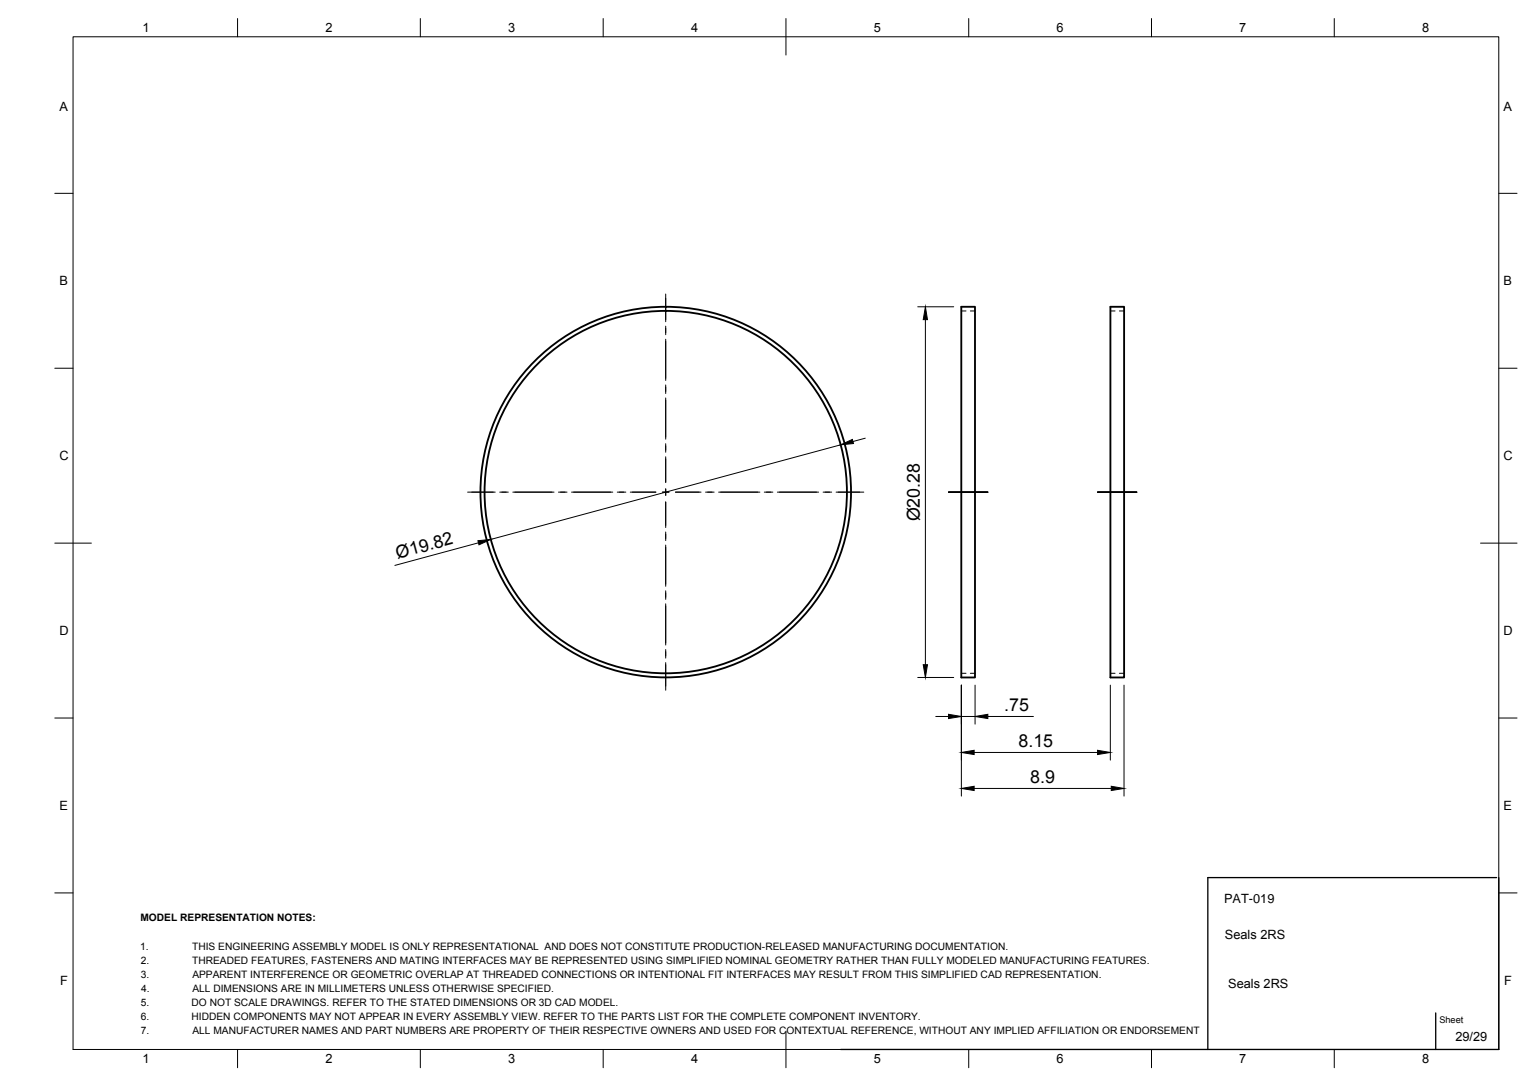
ISO-10303-21;
HEADER;
/* Generated by software containing ST-Developer
 * from STEP Tools, Inc. (www.steptools.com) 
 */

FILE_DESCRIPTION(
/* description */ ('Caster wheel assembly'),
/* implementation_level */ '2;1');

FILE_NAME(
/* name */ 'Seals 2RS.step',
/* time_stamp */ '2026-10-28T03:23:56-07:00',
/* author */ (''),
/* organization */ (''),
/* preprocessor_version */ 'ST-DEVELOPER v20.2',
/* originating_system */ 'Autodesk Translation Framework v15.17.0.0',
/* authorisation */ '');

FILE_SCHEMA (('AUTOMOTIVE_DESIGN { 1 0 10303 214 3 1 1 }'));
ENDSEC;

DATA;
#10=MECHANICAL_DESIGN_GEOMETRIC_PRESENTATION_REPRESENTATION('',(#250,#251),#5385);
#199=SHAPE_REPRESENTATION_RELATIONSHIP('SRR','None',#5497,#221);
#221=ADVANCED_BREP_SHAPE_REPRESENTATION('',(#279,#280),#5384);
#250=STYLED_ITEM('',(#5672),#279);
#251=STYLED_ITEM('',(#5672),#280);
#279=MANIFOLD_SOLID_BREP('Body1',#2678);
#280=MANIFOLD_SOLID_BREP('Body2',#2679);
#329=FACE_BOUND('',#798,.T.);
#330=FACE_BOUND('',#801,.T.);
#331=FACE_BOUND('',#804,.T.);
#332=FACE_BOUND('',#807,.T.);
#417=PLANE('',#3275);
#418=PLANE('',#3280);
#419=PLANE('',#3283);
#420=PLANE('',#3288);
#581=FACE_OUTER_BOUND('',#797,.T.);
#582=FACE_OUTER_BOUND('',#799,.T.);
#583=FACE_OUTER_BOUND('',#800,.T.);
#584=FACE_OUTER_BOUND('',#802,.T.);
#585=FACE_OUTER_BOUND('',#803,.T.);
#586=FACE_OUTER_BOUND('',#805,.T.);
#587=FACE_OUTER_BOUND('',#806,.T.);
#588=FACE_OUTER_BOUND('',#808,.T.);
#797=EDGE_LOOP('',(#2404));
#798=EDGE_LOOP('',(#2405));
#799=EDGE_LOOP('',(#2406,#2407,#2408,#2409));
#800=EDGE_LOOP('',(#2410));
#801=EDGE_LOOP('',(#2411));
#802=EDGE_LOOP('',(#2412,#2413,#2414,#2415));
#803=EDGE_LOOP('',(#2416));
#804=EDGE_LOOP('',(#2417));
#805=EDGE_LOOP('',(#2418,#2419,#2420,#2421));
#806=EDGE_LOOP('',(#2422));
#807=EDGE_LOOP('',(#2423));
#808=EDGE_LOOP('',(#2424,#2425,#2426,#2427));
#939=LINE('',#5297,#1073);
#940=LINE('',#5302,#1074);
#941=LINE('',#5311,#1075);
#942=LINE('',#5316,#1076);
#1073=VECTOR('',#4148,1.013815);
#1074=VECTOR('',#4155,0.991185);
#1075=VECTOR('',#4166,1.013815);
#1076=VECTOR('',#4173,0.991185);
#1228=CIRCLE('',#3276,1.013815);
#1229=CIRCLE('',#3277,0.991185);
#1230=CIRCLE('',#3279,1.013815);
#1231=CIRCLE('',#3281,0.991185);
#1232=CIRCLE('',#3284,1.013815);
#1233=CIRCLE('',#3285,0.991185);
#1234=CIRCLE('',#3287,1.013815);
#1235=CIRCLE('',#3289,0.991185);
#1451=VERTEX_POINT('',#5290);
#1452=VERTEX_POINT('',#5292);
#1453=VERTEX_POINT('',#5295);
#1454=VERTEX_POINT('',#5299);
#1455=VERTEX_POINT('',#5304);
#1456=VERTEX_POINT('',#5306);
#1457=VERTEX_POINT('',#5309);
#1458=VERTEX_POINT('',#5313);
#1770=EDGE_CURVE('',#1451,#1451,#1228,.T.);
#1771=EDGE_CURVE('',#1452,#1452,#1229,.T.);
#1772=EDGE_CURVE('',#1453,#1453,#1230,.T.);
#1773=EDGE_CURVE('',#1453,#1451,#939,.T.);
#1774=EDGE_CURVE('',#1454,#1454,#1231,.T.);
#1775=EDGE_CURVE('',#1454,#1452,#940,.T.);
#1776=EDGE_CURVE('',#1455,#1455,#1232,.T.);
#1777=EDGE_CURVE('',#1456,#1456,#1233,.T.);
#1778=EDGE_CURVE('',#1457,#1457,#1234,.T.);
#1779=EDGE_CURVE('',#1457,#1455,#941,.T.);
#1780=EDGE_CURVE('',#1458,#1458,#1235,.T.);
#1781=EDGE_CURVE('',#1458,#1456,#942,.T.);
#2404=ORIENTED_EDGE('',*,*,#1770,.F.);
#2405=ORIENTED_EDGE('',*,*,#1771,.T.);
#2406=ORIENTED_EDGE('',*,*,#1772,.F.);
#2407=ORIENTED_EDGE('',*,*,#1773,.T.);
#2408=ORIENTED_EDGE('',*,*,#1770,.T.);
#2409=ORIENTED_EDGE('',*,*,#1773,.F.);
#2410=ORIENTED_EDGE('',*,*,#1772,.T.);
#2411=ORIENTED_EDGE('',*,*,#1774,.F.);
#2412=ORIENTED_EDGE('',*,*,#1774,.T.);
#2413=ORIENTED_EDGE('',*,*,#1775,.T.);
#2414=ORIENTED_EDGE('',*,*,#1771,.F.);
#2415=ORIENTED_EDGE('',*,*,#1775,.F.);
#2416=ORIENTED_EDGE('',*,*,#1776,.F.);
#2417=ORIENTED_EDGE('',*,*,#1777,.T.);
#2418=ORIENTED_EDGE('',*,*,#1778,.F.);
#2419=ORIENTED_EDGE('',*,*,#1779,.T.);
#2420=ORIENTED_EDGE('',*,*,#1776,.T.);
#2421=ORIENTED_EDGE('',*,*,#1779,.F.);
#2422=ORIENTED_EDGE('',*,*,#1778,.T.);
#2423=ORIENTED_EDGE('',*,*,#1780,.F.);
#2424=ORIENTED_EDGE('',*,*,#1780,.T.);
#2425=ORIENTED_EDGE('',*,*,#1781,.T.);
#2426=ORIENTED_EDGE('',*,*,#1777,.F.);
#2427=ORIENTED_EDGE('',*,*,#1781,.F.);
#2477=CYLINDRICAL_SURFACE('',#3278,1.013815);
#2478=CYLINDRICAL_SURFACE('',#3282,0.991185);
#2479=CYLINDRICAL_SURFACE('',#3286,1.013815);
#2480=CYLINDRICAL_SURFACE('',#3290,0.991185);
#2641=ADVANCED_FACE('',(#581,#329),#417,.T.);
#2642=ADVANCED_FACE('',(#582),#2477,.T.);
#2643=ADVANCED_FACE('',(#583,#330),#418,.T.);
#2644=ADVANCED_FACE('',(#584),#2478,.F.);
#2645=ADVANCED_FACE('',(#585,#331),#419,.T.);
#2646=ADVANCED_FACE('',(#586),#2479,.T.);
#2647=ADVANCED_FACE('',(#587,#332),#420,.T.);
#2648=ADVANCED_FACE('',(#588),#2480,.F.);
#2678=CLOSED_SHELL('',(#2641,#2642,#2643,#2644));
#2679=CLOSED_SHELL('',(#2645,#2646,#2647,#2648));
#3274=AXIS2_PLACEMENT_3D('',#5288,#4136,#4137);
#3275=AXIS2_PLACEMENT_3D('',#5289,#4138,#4139);
#3276=AXIS2_PLACEMENT_3D('',#5291,#4140,#4141);
#3277=AXIS2_PLACEMENT_3D('',#5293,#4142,#4143);
#3278=AXIS2_PLACEMENT_3D('',#5294,#4144,#4145);
#3279=AXIS2_PLACEMENT_3D('',#5296,#4146,#4147);
#3280=AXIS2_PLACEMENT_3D('',#5298,#4149,#4150);
#3281=AXIS2_PLACEMENT_3D('',#5300,#4151,#4152);
#3282=AXIS2_PLACEMENT_3D('',#5301,#4153,#4154);
#3283=AXIS2_PLACEMENT_3D('',#5303,#4156,#4157);
#3284=AXIS2_PLACEMENT_3D('',#5305,#4158,#4159);
#3285=AXIS2_PLACEMENT_3D('',#5307,#4160,#4161);
#3286=AXIS2_PLACEMENT_3D('',#5308,#4162,#4163);
#3287=AXIS2_PLACEMENT_3D('',#5310,#4164,#4165);
#3288=AXIS2_PLACEMENT_3D('',#5312,#4167,#4168);
#3289=AXIS2_PLACEMENT_3D('',#5314,#4169,#4170);
#3290=AXIS2_PLACEMENT_3D('',#5315,#4171,#4172);
#4136=DIRECTION('axis',(0.,0.,1.));
#4137=DIRECTION('refdir',(1.,0.,0.));
#4138=DIRECTION('center_axis',(0.,1.,0.));
#4139=DIRECTION('ref_axis',(0.,0.,1.));
#4140=DIRECTION('center_axis',(0.,-1.,0.));
#4141=DIRECTION('ref_axis',(1.,0.,0.));
#4142=DIRECTION('center_axis',(0.,-1.,0.));
#4143=DIRECTION('ref_axis',(1.,0.,0.));
#4144=DIRECTION('center_axis',(0.,-1.,0.));
#4145=DIRECTION('ref_axis',(1.,0.,0.));
#4146=DIRECTION('center_axis',(0.,-1.,0.));
#4147=DIRECTION('ref_axis',(1.,0.,0.));
#4148=DIRECTION('',(0.,1.,0.));
#4149=DIRECTION('center_axis',(0.,-1.,0.));
#4150=DIRECTION('ref_axis',(0.,0.,-1.));
#4151=DIRECTION('center_axis',(0.,-1.,0.));
#4152=DIRECTION('ref_axis',(1.,0.,0.));
#4153=DIRECTION('center_axis',(0.,-1.,0.));
#4154=DIRECTION('ref_axis',(1.,0.,0.));
#4155=DIRECTION('',(0.,1.,0.));
#4156=DIRECTION('center_axis',(0.,1.,0.));
#4157=DIRECTION('ref_axis',(0.,0.,1.));
#4158=DIRECTION('center_axis',(0.,-1.,0.));
#4159=DIRECTION('ref_axis',(1.,0.,0.));
#4160=DIRECTION('center_axis',(0.,-1.,0.));
#4161=DIRECTION('ref_axis',(1.,0.,0.));
#4162=DIRECTION('center_axis',(0.,-1.,0.));
#4163=DIRECTION('ref_axis',(1.,0.,0.));
#4164=DIRECTION('center_axis',(0.,-1.,0.));
#4165=DIRECTION('ref_axis',(1.,0.,0.));
#4166=DIRECTION('',(0.,1.,0.));
#4167=DIRECTION('center_axis',(0.,-1.,0.));
#4168=DIRECTION('ref_axis',(0.,0.,-1.));
#4169=DIRECTION('center_axis',(0.,-1.,0.));
#4170=DIRECTION('ref_axis',(1.,0.,0.));
#4171=DIRECTION('center_axis',(0.,-1.,0.));
#4172=DIRECTION('ref_axis',(1.,0.,0.));
#4173=DIRECTION('',(0.,1.,0.));
#5288=CARTESIAN_POINT('',(0.,0.,0.));
#5289=CARTESIAN_POINT('Origin',(1.013815,0.445,0.));
#5290=CARTESIAN_POINT('',(-1.013815,0.445,-1.24156529467757E-16));
#5291=CARTESIAN_POINT('Origin',(0.,0.445,0.));
#5292=CARTESIAN_POINT('',(-0.991185,0.445,-1.21385153761287E-16));
#5293=CARTESIAN_POINT('Origin',(0.,0.445,0.));
#5294=CARTESIAN_POINT('Origin',(0.,0.4075,0.));
#5295=CARTESIAN_POINT('',(-1.013815,0.37,-1.24156529467757E-16));
#5296=CARTESIAN_POINT('Origin',(0.,0.37,0.));
#5297=CARTESIAN_POINT('',(-1.013815,0.4075,-1.24156529467757E-16));
#5298=CARTESIAN_POINT('Origin',(0.991185,0.37,0.));
#5299=CARTESIAN_POINT('',(-0.991185,0.37,-1.21385153761287E-16));
#5300=CARTESIAN_POINT('Origin',(0.,0.37,0.));
#5301=CARTESIAN_POINT('Origin',(0.,0.4075,0.));
#5302=CARTESIAN_POINT('',(-0.991185,0.4075,-1.21385153761287E-16));
#5303=CARTESIAN_POINT('Origin',(1.013815,-0.37,0.));
#5304=CARTESIAN_POINT('',(-1.013815,-0.37,-1.24156529467757E-16));
#5305=CARTESIAN_POINT('Origin',(0.,-0.37,0.));
#5306=CARTESIAN_POINT('',(-0.991185,-0.37,-1.21385153761287E-16));
#5307=CARTESIAN_POINT('Origin',(0.,-0.37,0.));
#5308=CARTESIAN_POINT('Origin',(0.,-0.4075,0.));
#5309=CARTESIAN_POINT('',(-1.013815,-0.445,-1.24156529467757E-16));
#5310=CARTESIAN_POINT('Origin',(0.,-0.445,0.));
#5311=CARTESIAN_POINT('',(-1.013815,-0.4075,-1.24156529467757E-16));
#5312=CARTESIAN_POINT('Origin',(0.991185,-0.445,0.));
#5313=CARTESIAN_POINT('',(-0.991185,-0.445,-1.21385153761287E-16));
#5314=CARTESIAN_POINT('Origin',(0.,-0.445,0.));
#5315=CARTESIAN_POINT('Origin',(0.,-0.4075,0.));
#5316=CARTESIAN_POINT('',(-0.991185,-0.4075,-1.21385153761287E-16));
#5356=UNCERTAINTY_MEASURE_WITH_UNIT(LENGTH_MEASURE(0.001),#5386,
'DISTANCE_ACCURACY_VALUE',
'Maximum model space distance between geometric entities at asserted c
onnectivities');
#5357=UNCERTAINTY_MEASURE_WITH_UNIT(LENGTH_MEASURE(0.001),#5386,
'DISTANCE_ACCURACY_VALUE',
'Maximum model space distance between geometric entities at asserted c
onnectivities');
#5384=(
GEOMETRIC_REPRESENTATION_CONTEXT(3)
GLOBAL_UNCERTAINTY_ASSIGNED_CONTEXT((#5356))
GLOBAL_UNIT_ASSIGNED_CONTEXT((#5386,#5388,#5389))
REPRESENTATION_CONTEXT('','3D')
);
#5385=(
GEOMETRIC_REPRESENTATION_CONTEXT(3)
GLOBAL_UNCERTAINTY_ASSIGNED_CONTEXT((#5357))
GLOBAL_UNIT_ASSIGNED_CONTEXT((#5386,#5388,#5389))
REPRESENTATION_CONTEXT('','3D')
);
#5386=(
LENGTH_UNIT()
NAMED_UNIT(*)
SI_UNIT(.CENTI.,.METRE.)
);
#5388=(
NAMED_UNIT(*)
PLANE_ANGLE_UNIT()
SI_UNIT($,.RADIAN.)
);
#5389=(
NAMED_UNIT(*)
SI_UNIT($,.STERADIAN.)
SOLID_ANGLE_UNIT()
);
#5416=SHAPE_DEFINITION_REPRESENTATION(#5457,#5497);
#5457=PRODUCT_DEFINITION_SHAPE('',$,#5525);
#5497=SHAPE_REPRESENTATION('',(#3274),#5384);
#5498=PRODUCT_DEFINITION_CONTEXT('part definition',#5581,'design');
#5525=PRODUCT_DEFINITION('Seals 2RS','Seals 2RS',#5552,#5498);
#5552=PRODUCT_DEFINITION_FORMATION('',$,#5609);
#5581=APPLICATION_CONTEXT(
'Core Data for Automotive Mechanical Design Process');
#5582=PRODUCT_CONTEXT('part definition',#5581,'mechanical');
#5609=PRODUCT('Seals 2RS','Seals 2RS','Seals 2RS',(#5582));
#5666=COLOUR_RGB('Grey',0.48,0.52,0.57);
#5667=FILL_AREA_STYLE_COLOUR('',#5666);
#5668=FILL_AREA_STYLE('',(#5667));
#5669=SURFACE_STYLE_FILL_AREA(#5668);
#5670=SURFACE_SIDE_STYLE('',(#5669));
#5671=SURFACE_STYLE_USAGE(.BOTH.,#5670);
#5672=PRESENTATION_STYLE_ASSIGNMENT((#5671));
ENDSEC;
END-ISO-10303-21;
